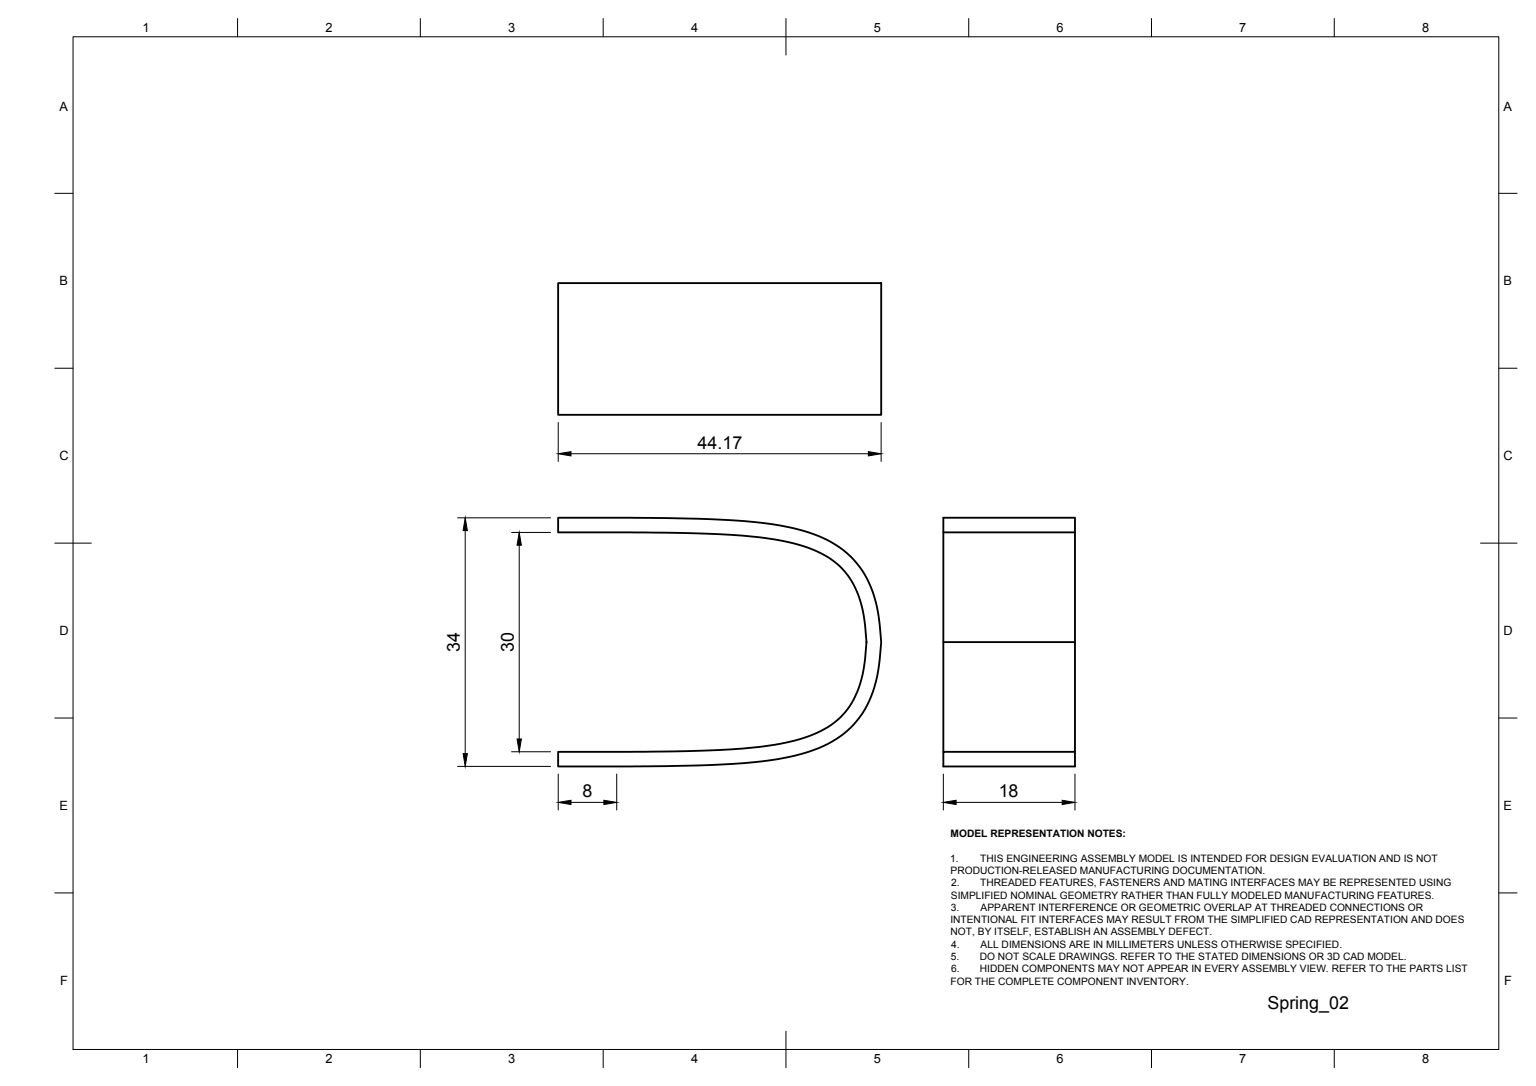
ISO-10303-21;
HEADER;
/* Generated by software containing ST-Developer
 * from STEP Tools, Inc. (www.steptools.com) 
 */

FILE_DESCRIPTION(
/* description */ (''),
/* implementation_level */ '2;1');

FILE_NAME(
/* name */ 'Spring_02.step',
/* time_stamp */ '2026-10-06T13:31:15-07:00',
/* author */ (''),
/* organization */ (''),
/* preprocessor_version */ 'ST-DEVELOPER v20.2',
/* originating_system */ 'Autodesk Translation Framework v15.15.0.0',
/* authorisation */ '');

FILE_SCHEMA (('AUTOMOTIVE_DESIGN { 1 0 10303 214 3 1 1 }'));
ENDSEC;

DATA;
#10=MECHANICAL_DESIGN_GEOMETRIC_PRESENTATION_REPRESENTATION('',(#81),#3154);
#51=B_SPLINE_SURFACE_WITH_KNOTS('',3,1,((#1764,#1765),(#1766,#1767),(#1768,
#1769),(#1770,#1771),(#1772,#1773),(#1774,#1775),(#1776,#1777),(#1778,#1779),
(#1780,#1781),(#1782,#1783),(#1784,#1785),(#1786,#1787),(#1788,#1789),(#1790,
#1791),(#1792,#1793),(#1794,#1795),(#1796,#1797),(#1798,#1799),(#1800,#1801)),
 .UNSPECIFIED.,.F.,.F.,.F.,(4,3,3,3,3,3,4),(2,2),(0.,0.25,0.625,0.869068416619454,
0.996324238316631,1.,1.10633190132162),(0.,2.16230058202055),
 .UNSPECIFIED.);
#52=B_SPLINE_SURFACE_WITH_KNOTS('',5,1,((#1843,#1844),(#1845,#1846),(#1847,
#1848),(#1849,#1850),(#1851,#1852),(#1853,#1854),(#1855,#1856),(#1857,#1858),
(#1859,#1860),(#1861,#1862),(#1863,#1864),(#1865,#1866),(#1867,#1868),(#1869,
#1870),(#1871,#1872),(#1873,#1874),(#1875,#1876),(#1877,#1878),(#1879,#1880),
(#1881,#1882),(#1883,#1884),(#1885,#1886),(#1887,#1888),(#1889,#1890),(#1891,
#1892)),.UNSPECIFIED.,.F.,.F.,.F.,(6,5,1,1,1,1,1,1,1,1,1,1,1,1,1,1,6),(2,
2),(-1.10044937423827,-1.,-0.933333333333333,-0.866666666666667,-0.8,-0.733333333333333,
-0.666666666666667,-0.6,-0.533333333333333,-0.466666666666667,-0.4,-0.333333333333333,
-0.266666666666667,-0.2,-0.133333333333333,-0.0666666666666667,0.),(0.,
2.16),.UNSPECIFIED.);
#53=B_SPLINE_SURFACE_WITH_KNOTS('',5,1,((#2046,#2047),(#2048,#2049),(#2050,
#2051),(#2052,#2053),(#2054,#2055),(#2056,#2057),(#2058,#2059),(#2060,#2061),
(#2062,#2063),(#2064,#2065),(#2066,#2067),(#2068,#2069),(#2070,#2071),(#2072,
#2073),(#2074,#2075),(#2076,#2077),(#2078,#2079),(#2080,#2081),(#2082,#2083),
(#2084,#2085),(#2086,#2087),(#2088,#2089),(#2090,#2091),(#2092,#2093),(#2094,
#2095)),.UNSPECIFIED.,.F.,.F.,.F.,(6,1,1,1,1,1,1,1,1,1,1,1,1,1,1,5,6),(2,
2),(0.,0.0666666666666667,0.133333333333333,0.2,0.266666666666667,0.333333333333333,
0.4,0.466666666666667,0.533333333333333,0.6,0.666666666666667,0.733333333333333,
0.8,0.866666666666667,0.933333333333333,1.,1.10044937423827),(0.,2.16),
 .UNSPECIFIED.);
#54=B_SPLINE_SURFACE_WITH_KNOTS('',3,1,((#2103,#2104),(#2105,#2106),(#2107,
#2108),(#2109,#2110),(#2111,#2112),(#2113,#2114),(#2115,#2116),(#2117,#2118),
(#2119,#2120),(#2121,#2122),(#2123,#2124),(#2125,#2126),(#2127,#2128),(#2129,
#2130),(#2131,#2132),(#2133,#2134),(#2135,#2136),(#2137,#2138),(#2139,#2140)),
 .UNSPECIFIED.,.F.,.F.,.F.,(4,3,3,3,3,3,4),(2,2),(-1.10633190132173,-1.,
-0.996324238316733,-0.869068416619454,-0.625,-0.25,0.),(0.,2.16230058202055),
 .UNSPECIFIED.);
#63=SHAPE_REPRESENTATION_RELATIONSHIP('SRR','None',#3191,#72);
#72=ADVANCED_BREP_SHAPE_REPRESENTATION('',(#90),#3147);
#81=STYLED_ITEM('',(#3243),#90);
#90=MANIFOLD_SOLID_BREP('Body1',#1083);
#102=PLANE('',#1213);
#103=PLANE('',#1214);
#104=PLANE('',#1215);
#105=PLANE('',#1216);
#106=PLANE('',#1217);
#107=PLANE('',#1218);
#108=PLANE('',#1219);
#109=PLANE('',#1220);
#182=FACE_OUTER_BOUND('',#246,.T.);
#183=FACE_OUTER_BOUND('',#247,.T.);
#184=FACE_OUTER_BOUND('',#248,.T.);
#185=FACE_OUTER_BOUND('',#249,.T.);
#186=FACE_OUTER_BOUND('',#250,.T.);
#187=FACE_OUTER_BOUND('',#251,.T.);
#188=FACE_OUTER_BOUND('',#252,.T.);
#189=FACE_OUTER_BOUND('',#253,.T.);
#190=FACE_OUTER_BOUND('',#254,.T.);
#191=FACE_OUTER_BOUND('',#255,.T.);
#192=FACE_OUTER_BOUND('',#256,.T.);
#193=FACE_OUTER_BOUND('',#257,.T.);
#246=EDGE_LOOP('',(#772,#773,#774,#775));
#247=EDGE_LOOP('',(#776,#777,#778,#779));
#248=EDGE_LOOP('',(#780,#781,#782,#783));
#249=EDGE_LOOP('',(#784,#785,#786,#787));
#250=EDGE_LOOP('',(#788,#789,#790,#791));
#251=EDGE_LOOP('',(#792,#793,#794,#795,#796,#797,#798,#799,#800,#801));
#252=EDGE_LOOP('',(#802,#803,#804,#805,#806,#807,#808,#809,#810,#811));
#253=EDGE_LOOP('',(#812,#813,#814,#815));
#254=EDGE_LOOP('',(#816,#817,#818,#819));
#255=EDGE_LOOP('',(#820,#821,#822,#823));
#256=EDGE_LOOP('',(#824,#825,#826,#827));
#257=EDGE_LOOP('',(#828,#829,#830,#831));
#308=LINE('',#1746,#374);
#309=LINE('',#1748,#375);
#310=LINE('',#1750,#376);
#311=LINE('',#1751,#377);
#312=LINE('',#1755,#378);
#313=LINE('',#1756,#379);
#314=LINE('',#1757,#380);
#315=LINE('',#1761,#381);
#316=LINE('',#1762,#382);
#317=LINE('',#1763,#383);
#318=LINE('',#1804,#384);
#319=LINE('',#1919,#385);
#320=LINE('',#1966,#386);
#321=LINE('',#1968,#387);
#322=LINE('',#1970,#388);
#323=LINE('',#2022,#389);
#324=LINE('',#2024,#390);
#325=LINE('',#2026,#391);
#326=LINE('',#2096,#392);
#327=LINE('',#2098,#393);
#328=LINE('',#2100,#394);
#329=LINE('',#2102,#395);
#374=VECTOR('',#1342,10.);
#375=VECTOR('',#1343,10.);
#376=VECTOR('',#1344,10.);
#377=VECTOR('',#1345,10.);
#378=VECTOR('',#1348,10.);
#379=VECTOR('',#1349,10.);
#380=VECTOR('',#1350,10.);
#381=VECTOR('',#1353,10.);
#382=VECTOR('',#1354,10.);
#383=VECTOR('',#1355,10.);
#384=VECTOR('',#1356,10.);
#385=VECTOR('',#1357,10.);
#386=VECTOR('',#1360,10.);
#387=VECTOR('',#1361,10.);
#388=VECTOR('',#1362,10.);
#389=VECTOR('',#1365,10.);
#390=VECTOR('',#1366,10.);
#391=VECTOR('',#1367,10.);
#392=VECTOR('',#1368,10.);
#393=VECTOR('',#1371,10.);
#394=VECTOR('',#1374,10.);
#395=VECTOR('',#1377,10.);
#442=B_SPLINE_CURVE_WITH_KNOTS('',3,(#1805,#1806,#1807,#1808,#1809,#1810,
#1811,#1812,#1813,#1814,#1815,#1816,#1817,#1818,#1819,#1820,#1821,#1822,
#1823),.UNSPECIFIED.,.F.,.F.,(4,3,3,3,3,3,4),(0.,0.25,0.625,0.869068416619454,
0.996324238316631,1.,1.03680973061555),.UNSPECIFIED.);
#443=B_SPLINE_CURVE_WITH_KNOTS('',3,(#1824,#1825,#1826,#1827,#1828,#1829,
#1830,#1831,#1832,#1833,#1834,#1835,#1836,#1837,#1838,#1839,#1840,#1841,
#1842),.UNSPECIFIED.,.F.,.F.,(4,3,3,3,3,3,4),(-1.03680973061555,-1.,-0.996324238316631,
-0.869068416619454,-0.625,-0.25,0.),.UNSPECIFIED.);
#444=B_SPLINE_CURVE_WITH_KNOTS('',5,(#1894,#1895,#1896,#1897,#1898,#1899,
#1900,#1901,#1902,#1903,#1904,#1905,#1906,#1907,#1908,#1909,#1910,#1911,
#1912,#1913,#1914,#1915,#1916,#1917),.UNSPECIFIED.,.F.,.F.,(6,1,1,1,1,1,
1,1,1,1,1,1,1,1,1,4,6),(0.,0.0666666666666667,0.133333333333333,0.2,0.266666666666667,
0.333333333333333,0.4,0.466666666666667,0.533333333333333,0.6,0.666666666666667,
0.733333333333333,0.8,0.866666666666667,0.933333333333333,1.,1.04017974969531),
 .UNSPECIFIED.);
#445=B_SPLINE_CURVE_WITH_KNOTS('',5,(#1920,#1921,#1922,#1923,#1924,#1925,
#1926,#1927,#1928,#1929,#1930,#1931,#1932,#1933,#1934,#1935,#1936,#1937,
#1938,#1939,#1940,#1941,#1942,#1943),.UNSPECIFIED.,.F.,.F.,(6,1,1,1,1,1,
1,1,1,1,1,1,1,1,1,4,6),(0.,0.0666666666666667,0.133333333333333,0.2,0.266666666666667,
0.333333333333333,0.4,0.466666666666667,0.533333333333333,0.6,0.666666666666667,
0.733333333333333,0.8,0.866666666666667,0.933333333333333,1.,1.04017974969531),
 .UNSPECIFIED.);
#446=B_SPLINE_CURVE_WITH_KNOTS('',3,(#1946,#1947,#1948,#1949,#1950,#1951,
#1952,#1953,#1954,#1955,#1956,#1957,#1958,#1959,#1960,#1961,#1962,#1963,
#1964),.UNSPECIFIED.,.F.,.F.,(4,3,3,3,3,3,4),(-1.03680973061555,-1.,-0.996324238316733,
-0.869068416619454,-0.625,-0.25,0.),.UNSPECIFIED.);
#447=B_SPLINE_CURVE_WITH_KNOTS('',5,(#1971,#1972,#1973,#1974,#1975,#1976,
#1977,#1978,#1979,#1980,#1981,#1982,#1983,#1984,#1985,#1986,#1987,#1988,
#1989,#1990,#1991,#1992,#1993,#1994),.UNSPECIFIED.,.F.,.F.,(6,4,1,1,1,1,
1,1,1,1,1,1,1,1,1,1,6),(-1.04017974969531,-1.,-0.933333333333333,-0.866666666666667,
-0.8,-0.733333333333333,-0.666666666666667,-0.6,-0.533333333333333,-0.466666666666667,
-0.4,-0.333333333333333,-0.266666666666667,-0.2,-0.133333333333333,-0.0666666666666667,
0.),.UNSPECIFIED.);
#448=B_SPLINE_CURVE_WITH_KNOTS('',5,(#1997,#1998,#1999,#2000,#2001,#2002,
#2003,#2004,#2005,#2006,#2007,#2008,#2009,#2010,#2011,#2012,#2013,#2014,
#2015,#2016,#2017,#2018,#2019,#2020),.UNSPECIFIED.,.F.,.F.,(6,4,1,1,1,1,
1,1,1,1,1,1,1,1,1,1,6),(-1.04017974969531,-1.,-0.933333333333333,-0.866666666666667,
-0.8,-0.733333333333333,-0.666666666666667,-0.6,-0.533333333333333,-0.466666666666667,
-0.4,-0.333333333333333,-0.266666666666667,-0.2,-0.133333333333333,-0.0666666666666667,
0.),.UNSPECIFIED.);
#449=B_SPLINE_CURVE_WITH_KNOTS('',3,(#2027,#2028,#2029,#2030,#2031,#2032,
#2033,#2034,#2035,#2036,#2037,#2038,#2039,#2040,#2041,#2042,#2043,#2044,
#2045),.UNSPECIFIED.,.F.,.F.,(4,3,3,3,3,3,4),(0.,0.25,0.625,0.869068416619454,
0.996324238316733,1.,1.03680973061555),.UNSPECIFIED.);
#496=VERTEX_POINT('',#1744);
#497=VERTEX_POINT('',#1745);
#498=VERTEX_POINT('',#1747);
#499=VERTEX_POINT('',#1749);
#500=VERTEX_POINT('',#1753);
#501=VERTEX_POINT('',#1754);
#502=VERTEX_POINT('',#1759);
#503=VERTEX_POINT('',#1760);
#504=VERTEX_POINT('',#1802);
#505=VERTEX_POINT('',#1803);
#506=VERTEX_POINT('',#1893);
#507=VERTEX_POINT('',#1918);
#508=VERTEX_POINT('',#1945);
#509=VERTEX_POINT('',#1965);
#510=VERTEX_POINT('',#1967);
#511=VERTEX_POINT('',#1969);
#512=VERTEX_POINT('',#1996);
#513=VERTEX_POINT('',#2021);
#514=VERTEX_POINT('',#2023);
#515=VERTEX_POINT('',#2025);
#602=EDGE_CURVE('',#496,#497,#308,.T.);
#603=EDGE_CURVE('',#498,#497,#309,.T.);
#604=EDGE_CURVE('',#498,#499,#310,.T.);
#605=EDGE_CURVE('',#496,#499,#311,.T.);
#606=EDGE_CURVE('',#500,#501,#312,.T.);
#607=EDGE_CURVE('',#497,#501,#313,.T.);
#608=EDGE_CURVE('',#500,#496,#314,.T.);
#609=EDGE_CURVE('',#502,#503,#315,.T.);
#610=EDGE_CURVE('',#501,#503,#316,.T.);
#611=EDGE_CURVE('',#502,#500,#317,.T.);
#612=EDGE_CURVE('',#504,#505,#318,.F.);
#613=EDGE_CURVE('',#503,#505,#442,.T.);
#614=EDGE_CURVE('',#504,#502,#443,.T.);
#615=EDGE_CURVE('',#506,#498,#444,.F.);
#616=EDGE_CURVE('',#507,#506,#319,.F.);
#617=EDGE_CURVE('',#499,#507,#445,.T.);
#618=EDGE_CURVE('',#505,#508,#446,.T.);
#619=EDGE_CURVE('',#508,#509,#320,.T.);
#620=EDGE_CURVE('',#509,#510,#321,.T.);
#621=EDGE_CURVE('',#510,#511,#322,.T.);
#622=EDGE_CURVE('',#511,#506,#447,.F.);
#623=EDGE_CURVE('',#507,#512,#448,.T.);
#624=EDGE_CURVE('',#512,#513,#323,.T.);
#625=EDGE_CURVE('',#513,#514,#324,.T.);
#626=EDGE_CURVE('',#514,#515,#325,.T.);
#627=EDGE_CURVE('',#515,#504,#449,.T.);
#628=EDGE_CURVE('',#512,#511,#326,.T.);
#629=EDGE_CURVE('',#513,#510,#327,.T.);
#630=EDGE_CURVE('',#514,#509,#328,.T.);
#631=EDGE_CURVE('',#515,#508,#329,.T.);
#772=ORIENTED_EDGE('',*,*,#602,.T.);
#773=ORIENTED_EDGE('',*,*,#603,.F.);
#774=ORIENTED_EDGE('',*,*,#604,.T.);
#775=ORIENTED_EDGE('',*,*,#605,.F.);
#776=ORIENTED_EDGE('',*,*,#606,.T.);
#777=ORIENTED_EDGE('',*,*,#607,.F.);
#778=ORIENTED_EDGE('',*,*,#602,.F.);
#779=ORIENTED_EDGE('',*,*,#608,.F.);
#780=ORIENTED_EDGE('',*,*,#609,.T.);
#781=ORIENTED_EDGE('',*,*,#610,.F.);
#782=ORIENTED_EDGE('',*,*,#606,.F.);
#783=ORIENTED_EDGE('',*,*,#611,.F.);
#784=ORIENTED_EDGE('',*,*,#612,.T.);
#785=ORIENTED_EDGE('',*,*,#613,.F.);
#786=ORIENTED_EDGE('',*,*,#609,.F.);
#787=ORIENTED_EDGE('',*,*,#614,.F.);
#788=ORIENTED_EDGE('',*,*,#604,.F.);
#789=ORIENTED_EDGE('',*,*,#615,.F.);
#790=ORIENTED_EDGE('',*,*,#616,.F.);
#791=ORIENTED_EDGE('',*,*,#617,.F.);
#792=ORIENTED_EDGE('',*,*,#618,.T.);
#793=ORIENTED_EDGE('',*,*,#619,.T.);
#794=ORIENTED_EDGE('',*,*,#620,.T.);
#795=ORIENTED_EDGE('',*,*,#621,.T.);
#796=ORIENTED_EDGE('',*,*,#622,.T.);
#797=ORIENTED_EDGE('',*,*,#615,.T.);
#798=ORIENTED_EDGE('',*,*,#603,.T.);
#799=ORIENTED_EDGE('',*,*,#607,.T.);
#800=ORIENTED_EDGE('',*,*,#610,.T.);
#801=ORIENTED_EDGE('',*,*,#613,.T.);
#802=ORIENTED_EDGE('',*,*,#623,.T.);
#803=ORIENTED_EDGE('',*,*,#624,.T.);
#804=ORIENTED_EDGE('',*,*,#625,.T.);
#805=ORIENTED_EDGE('',*,*,#626,.T.);
#806=ORIENTED_EDGE('',*,*,#627,.T.);
#807=ORIENTED_EDGE('',*,*,#614,.T.);
#808=ORIENTED_EDGE('',*,*,#611,.T.);
#809=ORIENTED_EDGE('',*,*,#608,.T.);
#810=ORIENTED_EDGE('',*,*,#605,.T.);
#811=ORIENTED_EDGE('',*,*,#617,.T.);
#812=ORIENTED_EDGE('',*,*,#616,.T.);
#813=ORIENTED_EDGE('',*,*,#622,.F.);
#814=ORIENTED_EDGE('',*,*,#628,.F.);
#815=ORIENTED_EDGE('',*,*,#623,.F.);
#816=ORIENTED_EDGE('',*,*,#628,.T.);
#817=ORIENTED_EDGE('',*,*,#621,.F.);
#818=ORIENTED_EDGE('',*,*,#629,.F.);
#819=ORIENTED_EDGE('',*,*,#624,.F.);
#820=ORIENTED_EDGE('',*,*,#629,.T.);
#821=ORIENTED_EDGE('',*,*,#620,.F.);
#822=ORIENTED_EDGE('',*,*,#630,.F.);
#823=ORIENTED_EDGE('',*,*,#625,.F.);
#824=ORIENTED_EDGE('',*,*,#630,.T.);
#825=ORIENTED_EDGE('',*,*,#619,.F.);
#826=ORIENTED_EDGE('',*,*,#631,.F.);
#827=ORIENTED_EDGE('',*,*,#626,.F.);
#828=ORIENTED_EDGE('',*,*,#631,.T.);
#829=ORIENTED_EDGE('',*,*,#618,.F.);
#830=ORIENTED_EDGE('',*,*,#612,.F.);
#831=ORIENTED_EDGE('',*,*,#627,.F.);
#1033=ADVANCED_FACE('',(#182),#102,.T.);
#1034=ADVANCED_FACE('',(#183),#103,.T.);
#1035=ADVANCED_FACE('',(#184),#104,.T.);
#1036=ADVANCED_FACE('',(#185),#51,.T.);
#1037=ADVANCED_FACE('',(#186),#52,.T.);
#1038=ADVANCED_FACE('',(#187),#105,.T.);
#1039=ADVANCED_FACE('',(#188),#106,.F.);
#1040=ADVANCED_FACE('',(#189),#53,.T.);
#1041=ADVANCED_FACE('',(#190),#107,.T.);
#1042=ADVANCED_FACE('',(#191),#108,.T.);
#1043=ADVANCED_FACE('',(#192),#109,.T.);
#1044=ADVANCED_FACE('',(#193),#54,.T.);
#1083=CLOSED_SHELL('',(#1033,#1034,#1035,#1036,#1037,#1038,#1039,#1040,
#1041,#1042,#1043,#1044));
#1212=AXIS2_PLACEMENT_3D('',#1742,#1338,#1339);
#1213=AXIS2_PLACEMENT_3D('',#1743,#1340,#1341);
#1214=AXIS2_PLACEMENT_3D('',#1752,#1346,#1347);
#1215=AXIS2_PLACEMENT_3D('',#1758,#1351,#1352);
#1216=AXIS2_PLACEMENT_3D('',#1944,#1358,#1359);
#1217=AXIS2_PLACEMENT_3D('',#1995,#1363,#1364);
#1218=AXIS2_PLACEMENT_3D('',#2097,#1369,#1370);
#1219=AXIS2_PLACEMENT_3D('',#2099,#1372,#1373);
#1220=AXIS2_PLACEMENT_3D('',#2101,#1375,#1376);
#1338=DIRECTION('axis',(0.,0.,1.));
#1339=DIRECTION('refdir',(1.,0.,0.));
#1340=DIRECTION('center_axis',(-1.,0.,0.));
#1341=DIRECTION('ref_axis',(0.,0.,1.));
#1342=DIRECTION('',(0.,1.,0.));
#1343=DIRECTION('',(0.,0.,1.));
#1344=DIRECTION('',(0.,-1.,0.));
#1345=DIRECTION('',(0.,0.,-1.));
#1346=DIRECTION('center_axis',(0.,0.,1.));
#1347=DIRECTION('ref_axis',(1.,0.,0.));
#1348=DIRECTION('',(0.,1.,0.));
#1349=DIRECTION('',(1.,0.,0.));
#1350=DIRECTION('',(-1.,0.,0.));
#1351=DIRECTION('center_axis',(1.,0.,0.));
#1352=DIRECTION('ref_axis',(0.,0.,-1.));
#1353=DIRECTION('',(0.,1.,0.));
#1354=DIRECTION('',(0.,0.,-1.));
#1355=DIRECTION('',(0.,0.,1.));
#1356=DIRECTION('',(0.,-1.,0.));
#1357=DIRECTION('',(0.,-1.,0.));
#1358=DIRECTION('center_axis',(0.,1.,0.));
#1359=DIRECTION('ref_axis',(1.,0.,0.));
#1360=DIRECTION('',(0.,0.,1.));
#1361=DIRECTION('',(1.,0.,0.));
#1362=DIRECTION('',(0.,0.,-1.));
#1363=DIRECTION('center_axis',(0.,1.,0.));
#1364=DIRECTION('ref_axis',(1.,0.,0.));
#1365=DIRECTION('',(0.,0.,1.));
#1366=DIRECTION('',(-1.,0.,0.));
#1367=DIRECTION('',(0.,0.,-1.));
#1368=DIRECTION('',(0.,1.,0.));
#1369=DIRECTION('center_axis',(1.,0.,0.));
#1370=DIRECTION('ref_axis',(0.,0.,-1.));
#1371=DIRECTION('',(0.,1.,0.));
#1372=DIRECTION('center_axis',(0.,0.,1.));
#1373=DIRECTION('ref_axis',(1.,0.,0.));
#1374=DIRECTION('',(0.,1.,0.));
#1375=DIRECTION('center_axis',(-1.,0.,0.));
#1376=DIRECTION('ref_axis',(0.,0.,1.));
#1377=DIRECTION('',(0.,1.,0.));
#1742=CARTESIAN_POINT('',(0.,0.,0.));
#1743=CARTESIAN_POINT('Origin',(-17.,0.,316.));
#1744=CARTESIAN_POINT('',(-17.,-9.,324.));
#1745=CARTESIAN_POINT('',(-17.,9.,324.));
#1746=CARTESIAN_POINT('',(-17.,0.,324.));
#1747=CARTESIAN_POINT('',(-17.,9.,316.));
#1748=CARTESIAN_POINT('',(-17.,9.,324.));
#1749=CARTESIAN_POINT('',(-17.,-9.,316.));
#1750=CARTESIAN_POINT('',(-17.,0.,316.));
#1751=CARTESIAN_POINT('',(-17.,-9.,324.));
#1752=CARTESIAN_POINT('Origin',(-17.,0.,324.));
#1753=CARTESIAN_POINT('',(-15.,-9.,324.));
#1754=CARTESIAN_POINT('',(-15.,9.,324.));
#1755=CARTESIAN_POINT('',(-15.,0.,324.));
#1756=CARTESIAN_POINT('',(-17.,9.,324.));
#1757=CARTESIAN_POINT('',(-17.,-9.,324.));
#1758=CARTESIAN_POINT('Origin',(-15.,0.,324.));
#1759=CARTESIAN_POINT('',(-15.,-9.,316.));
#1760=CARTESIAN_POINT('',(-15.,9.,316.));
#1761=CARTESIAN_POINT('',(-15.,0.,316.));
#1762=CARTESIAN_POINT('',(-15.,9.,324.));
#1763=CARTESIAN_POINT('',(-15.,-9.,324.));
#1764=CARTESIAN_POINT('Ctrl Pts',(-15.,-9.01917151683795,316.));
#1765=CARTESIAN_POINT('Ctrl Pts',(-15.,12.6038343033676,316.));
#1766=CARTESIAN_POINT('Ctrl Pts',(-15.,-9.01917151683795,312.917218954967));
#1767=CARTESIAN_POINT('Ctrl Pts',(-15.,12.6038343033676,312.917218954967));
#1768=CARTESIAN_POINT('Ctrl Pts',(-14.9804665025967,-9.01917151683795,309.284971969759));
#1769=CARTESIAN_POINT('Ctrl Pts',(-14.9804665025967,12.6038343033676,309.284971969759));
#1770=CARTESIAN_POINT('Ctrl Pts',(-14.8743203079702,-9.01917151683795,305.389849883143));
#1771=CARTESIAN_POINT('Ctrl Pts',(-14.8743203079702,12.6038343033676,305.389849883143));
#1772=CARTESIAN_POINT('Ctrl Pts',(-14.7151010160305,-9.01917151683795,299.547166753218));
#1773=CARTESIAN_POINT('Ctrl Pts',(-14.7151010160305,12.6038343033676,299.547166753218));
#1774=CARTESIAN_POINT('Ctrl Pts',(-14.3613339472215,-9.01917151683795,293.114195242939));
#1775=CARTESIAN_POINT('Ctrl Pts',(-14.3613339472215,12.6038343033676,293.114195242939));
#1776=CARTESIAN_POINT('Ctrl Pts',(-12.5329121501934,-9.01917151683795,288.887907445925));
#1777=CARTESIAN_POINT('Ctrl Pts',(-12.5329121501934,12.6038343033676,288.887907445925));
#1778=CARTESIAN_POINT('Ctrl Pts',(-11.3428854490917,-9.01917151683795,286.13723179047));
#1779=CARTESIAN_POINT('Ctrl Pts',(-11.3428854490917,12.6038343033676,286.13723179047));
#1780=CARTESIAN_POINT('Ctrl Pts',(-9.6259837213127,-9.01917151683795,284.320800585332));
#1781=CARTESIAN_POINT('Ctrl Pts',(-9.6259837213127,12.6038343033676,284.320800585332));
#1782=CARTESIAN_POINT('Ctrl Pts',(-6.96718239188881,-9.01917151683795,283.179505866003));
#1783=CARTESIAN_POINT('Ctrl Pts',(-6.96718239188881,12.6038343033676,283.179505866003));
#1784=CARTESIAN_POINT('Ctrl Pts',(-5.58089918248474,-9.01917151683795,282.584441583133));
#1785=CARTESIAN_POINT('Ctrl Pts',(-5.58089918248474,12.6038343033676,282.584441583133));
#1786=CARTESIAN_POINT('Ctrl Pts',(-3.9277760249776,-9.01917151683795,282.184209001161));
#1787=CARTESIAN_POINT('Ctrl Pts',(-3.9277760249776,12.6038343033676,282.184209001161));
#1788=CARTESIAN_POINT('Ctrl Pts',(-2.00000000000228,-9.01917151683795,282.007690234858));
#1789=CARTESIAN_POINT('Ctrl Pts',(-2.00000000000228,12.6038343033676,282.007690234858));
#1790=CARTESIAN_POINT('Ctrl Pts',(-1.94431052069769,-9.01917151683795,282.002590971222));
#1791=CARTESIAN_POINT('Ctrl Pts',(-1.94431052069769,12.6038343033676,282.002590971222));
#1792=CARTESIAN_POINT('Ctrl Pts',(-1.88839473154277,-9.01917151683795,281.997678278411));
#1793=CARTESIAN_POINT('Ctrl Pts',(-1.88839473154277,12.6038343033676,281.997678278411));
#1794=CARTESIAN_POINT('Ctrl Pts',(-1.8322528584517,-9.01917151683795,281.992952808398));
#1795=CARTESIAN_POINT('Ctrl Pts',(-1.8322528584517,12.6038343033676,281.992952808398));
#1796=CARTESIAN_POINT('Ctrl Pts',(-0.067982678772372,-9.01917151683795,
281.844453918553));
#1797=CARTESIAN_POINT('Ctrl Pts',(-0.067982678772372,12.6038343033676,281.844453918553));
#1798=CARTESIAN_POINT('Ctrl Pts',(1.69628750090713,-9.01917151683795,281.695955028709));
#1799=CARTESIAN_POINT('Ctrl Pts',(1.69628750090713,12.6038343033676,281.695955028709));
#1800=CARTESIAN_POINT('Ctrl Pts',(3.46055768058644,-9.01917151683795,281.547456138864));
#1801=CARTESIAN_POINT('Ctrl Pts',(3.46055768058644,12.6038343033676,281.547456138864));
#1802=CARTESIAN_POINT('',(-2.61075883134509E-14,-9.,281.838731806123));
#1803=CARTESIAN_POINT('',(-2.61075883134509E-14,9.,281.838731806123));
#1804=CARTESIAN_POINT('',(-5.91540705308091E-14,9.,281.838731806123));
#1805=CARTESIAN_POINT('Ctrl Pts',(-15.,9.,316.));
#1806=CARTESIAN_POINT('Ctrl Pts',(-15.,9.,312.917218954967));
#1807=CARTESIAN_POINT('Ctrl Pts',(-14.9804665025967,9.,309.284971969759));
#1808=CARTESIAN_POINT('Ctrl Pts',(-14.8743203079702,9.,305.389849883143));
#1809=CARTESIAN_POINT('Ctrl Pts',(-14.7151010160305,9.,299.547166753218));
#1810=CARTESIAN_POINT('Ctrl Pts',(-14.3613339472215,9.,293.114195242939));
#1811=CARTESIAN_POINT('Ctrl Pts',(-12.5329121501934,9.,288.887907445925));
#1812=CARTESIAN_POINT('Ctrl Pts',(-11.3428854490917,9.,286.13723179047));
#1813=CARTESIAN_POINT('Ctrl Pts',(-9.6259837213127,9.,284.320800585332));
#1814=CARTESIAN_POINT('Ctrl Pts',(-6.96718239188881,9.,283.179505866003));
#1815=CARTESIAN_POINT('Ctrl Pts',(-5.58089918248474,9.,282.584441583133));
#1816=CARTESIAN_POINT('Ctrl Pts',(-3.9277760249776,9.,282.184209001161));
#1817=CARTESIAN_POINT('Ctrl Pts',(-2.00000000000228,9.,282.007690234858));
#1818=CARTESIAN_POINT('Ctrl Pts',(-1.94431052069769,9.,282.002590971222));
#1819=CARTESIAN_POINT('Ctrl Pts',(-1.88839473154277,9.,281.997678278411));
#1820=CARTESIAN_POINT('Ctrl Pts',(-1.8322528584517,9.,281.992952808398));
#1821=CARTESIAN_POINT('Ctrl Pts',(-1.22150190563454,9.,281.941545807639));
#1822=CARTESIAN_POINT('Ctrl Pts',(-0.610750952817352,9.,281.890138806881));
#1823=CARTESIAN_POINT('Ctrl Pts',(-1.61426427780498E-13,9.,281.838731806122));
#1824=CARTESIAN_POINT('Ctrl Pts',(-1.39499523044151E-13,-9.,281.838731806122));
#1825=CARTESIAN_POINT('Ctrl Pts',(-0.610750952817337,-9.,281.890138806881));
#1826=CARTESIAN_POINT('Ctrl Pts',(-1.22150190563453,-9.,281.941545807639));
#1827=CARTESIAN_POINT('Ctrl Pts',(-1.8322528584517,-9.,281.992952808398));
#1828=CARTESIAN_POINT('Ctrl Pts',(-1.88839473154277,-9.,281.997678278411));
#1829=CARTESIAN_POINT('Ctrl Pts',(-1.94431052069769,-9.,282.002590971222));
#1830=CARTESIAN_POINT('Ctrl Pts',(-2.00000000000228,-9.,282.007690234858));
#1831=CARTESIAN_POINT('Ctrl Pts',(-3.9277760249776,-9.,282.184209001161));
#1832=CARTESIAN_POINT('Ctrl Pts',(-5.58089918248474,-9.,282.584441583133));
#1833=CARTESIAN_POINT('Ctrl Pts',(-6.96718239188881,-9.,283.179505866003));
#1834=CARTESIAN_POINT('Ctrl Pts',(-9.6259837213127,-9.,284.320800585332));
#1835=CARTESIAN_POINT('Ctrl Pts',(-11.3428854490917,-9.,286.13723179047));
#1836=CARTESIAN_POINT('Ctrl Pts',(-12.5329121501934,-9.,288.887907445925));
#1837=CARTESIAN_POINT('Ctrl Pts',(-14.3613339472215,-9.,293.114195242939));
#1838=CARTESIAN_POINT('Ctrl Pts',(-14.7151010160305,-9.,299.547166753218));
#1839=CARTESIAN_POINT('Ctrl Pts',(-14.8743203079702,-9.,305.389849883143));
#1840=CARTESIAN_POINT('Ctrl Pts',(-14.9804665025967,-9.,309.284971969759));
#1841=CARTESIAN_POINT('Ctrl Pts',(-15.,-9.,312.917218954967));
#1842=CARTESIAN_POINT('Ctrl Pts',(-15.,-9.,316.));
#1843=CARTESIAN_POINT('Ctrl Pts',(3.,-9.,279.579149238152));
#1844=CARTESIAN_POINT('Ctrl Pts',(3.,12.6,279.579149238152));
#1845=CARTESIAN_POINT('Ctrl Pts',(2.,-9.,279.663319390522));
#1846=CARTESIAN_POINT('Ctrl Pts',(2.,12.6,279.663319390522));
#1847=CARTESIAN_POINT('Ctrl Pts',(1.,-9.,279.747489542891));
#1848=CARTESIAN_POINT('Ctrl Pts',(1.,12.6,279.747489542891));
#1849=CARTESIAN_POINT('Ctrl Pts',(-5.55111512312578E-16,-9.,279.831659695261));
#1850=CARTESIAN_POINT('Ctrl Pts',(-5.55111512312578E-16,12.6,279.831659695261));
#1851=CARTESIAN_POINT('Ctrl Pts',(-1.,-9.,279.91582984763));
#1852=CARTESIAN_POINT('Ctrl Pts',(-1.,12.6,279.91582984763));
#1853=CARTESIAN_POINT('Ctrl Pts',(-2.,-9.,280.));
#1854=CARTESIAN_POINT('Ctrl Pts',(-2.,12.6,280.));
#1855=CARTESIAN_POINT('Ctrl Pts',(-2.66368424066569,-9.,280.055862403662));
#1856=CARTESIAN_POINT('Ctrl Pts',(-2.66368424066569,12.6,280.055862403662));
#1857=CARTESIAN_POINT('Ctrl Pts',(-3.9517913938126,-9.,280.208504145521));
#1858=CARTESIAN_POINT('Ctrl Pts',(-3.9517913938126,12.6,280.208504145521));
#1859=CARTESIAN_POINT('Ctrl Pts',(-5.76616670029465,-9.,280.560219196132));
#1860=CARTESIAN_POINT('Ctrl Pts',(-5.76616670029465,12.6,280.560219196132));
#1861=CARTESIAN_POINT('Ctrl Pts',(-7.94806288019228,-9.,281.276448102944));
#1862=CARTESIAN_POINT('Ctrl Pts',(-7.94806288019228,12.6,281.276448102944));
#1863=CARTESIAN_POINT('Ctrl Pts',(-10.2723403348262,-9.,282.590975648728));
#1864=CARTESIAN_POINT('Ctrl Pts',(-10.2723403348262,12.6,282.590975648728));
#1865=CARTESIAN_POINT('Ctrl Pts',(-12.1890242800701,-9.,284.326851421562));
#1866=CARTESIAN_POINT('Ctrl Pts',(-12.1890242800701,12.6,284.326851421562));
#1867=CARTESIAN_POINT('Ctrl Pts',(-13.7033484644208,-9.,286.473438815185));
#1868=CARTESIAN_POINT('Ctrl Pts',(-13.7033484644208,12.6,286.473438815185));
#1869=CARTESIAN_POINT('Ctrl Pts',(-14.8403951587419,-9.,288.995763819941));
#1870=CARTESIAN_POINT('Ctrl Pts',(-14.8403951587419,12.6,288.995763819941));
#1871=CARTESIAN_POINT('Ctrl Pts',(-15.6496061172615,-9.,291.82914277586));
#1872=CARTESIAN_POINT('Ctrl Pts',(-15.6496061172615,12.6,291.82914277586));
#1873=CARTESIAN_POINT('Ctrl Pts',(-16.1926929497518,-9.,294.892205598351));
#1874=CARTESIAN_POINT('Ctrl Pts',(-16.1926929497518,12.6,294.892205598351));
#1875=CARTESIAN_POINT('Ctrl Pts',(-16.5359735439045,-9.,298.095070696299));
#1876=CARTESIAN_POINT('Ctrl Pts',(-16.5359735439045,12.6,298.095070696299));
#1877=CARTESIAN_POINT('Ctrl Pts',(-16.7422790149997,-9.,301.348120547886));
#1878=CARTESIAN_POINT('Ctrl Pts',(-16.7422790149997,12.6,301.348120547886));
#1879=CARTESIAN_POINT('Ctrl Pts',(-16.8634487703245,-9.,304.57015716772));
#1880=CARTESIAN_POINT('Ctrl Pts',(-16.8634487703245,12.6,304.57015716772));
#1881=CARTESIAN_POINT('Ctrl Pts',(-16.9338349467122,-9.,307.69587590639));
#1882=CARTESIAN_POINT('Ctrl Pts',(-16.9338349467122,12.6,307.69587590639));
#1883=CARTESIAN_POINT('Ctrl Pts',(-16.9745170477256,-9.,310.674187150777));
#1884=CARTESIAN_POINT('Ctrl Pts',(-16.9745170477256,12.6,310.674187150777));
#1885=CARTESIAN_POINT('Ctrl Pts',(-16.9920318646118,-9.,312.909176752281));
#1886=CARTESIAN_POINT('Ctrl Pts',(-16.9920318646118,12.6,312.909176752281));
#1887=CARTESIAN_POINT('Ctrl Pts',(-16.9985513080952,-9.,314.491917916066));
#1888=CARTESIAN_POINT('Ctrl Pts',(-16.9985513080952,12.6,314.491917916066));
#1889=CARTESIAN_POINT('Ctrl Pts',(-17.,-9.,315.50441646936));
#1890=CARTESIAN_POINT('Ctrl Pts',(-17.,12.6,315.50441646936));
#1891=CARTESIAN_POINT('Ctrl Pts',(-17.,-9.,316.));
#1892=CARTESIAN_POINT('Ctrl Pts',(-17.,12.6,316.));
#1893=CARTESIAN_POINT('',(-1.13335267097151E-15,9.,279.831659695261));
#1894=CARTESIAN_POINT('Ctrl Pts',(-17.,9.,316.));
#1895=CARTESIAN_POINT('Ctrl Pts',(-17.,9.,315.50441646936));
#1896=CARTESIAN_POINT('Ctrl Pts',(-16.9985513080952,9.,314.491917916066));
#1897=CARTESIAN_POINT('Ctrl Pts',(-16.9920318646118,9.,312.909176752281));
#1898=CARTESIAN_POINT('Ctrl Pts',(-16.9745170477256,9.,310.674187150777));
#1899=CARTESIAN_POINT('Ctrl Pts',(-16.9338349467122,9.,307.69587590639));
#1900=CARTESIAN_POINT('Ctrl Pts',(-16.8634487703245,9.,304.57015716772));
#1901=CARTESIAN_POINT('Ctrl Pts',(-16.7422790149997,9.,301.348120547886));
#1902=CARTESIAN_POINT('Ctrl Pts',(-16.5359735439045,9.,298.095070696299));
#1903=CARTESIAN_POINT('Ctrl Pts',(-16.1926929497518,9.,294.892205598351));
#1904=CARTESIAN_POINT('Ctrl Pts',(-15.6496061172615,9.,291.82914277586));
#1905=CARTESIAN_POINT('Ctrl Pts',(-14.8403951587419,9.,288.995763819941));
#1906=CARTESIAN_POINT('Ctrl Pts',(-13.7033484644208,9.,286.473438815185));
#1907=CARTESIAN_POINT('Ctrl Pts',(-12.1890242800701,9.,284.326851421562));
#1908=CARTESIAN_POINT('Ctrl Pts',(-10.2723403348262,9.,282.590975648728));
#1909=CARTESIAN_POINT('Ctrl Pts',(-7.94806288019228,9.,281.276448102944));
#1910=CARTESIAN_POINT('Ctrl Pts',(-5.76616670029465,9.,280.560219196132));
#1911=CARTESIAN_POINT('Ctrl Pts',(-3.9517913938126,9.,280.208504145521));
#1912=CARTESIAN_POINT('Ctrl Pts',(-2.66368424066569,9.,280.055862403662));
#1913=CARTESIAN_POINT('Ctrl Pts',(-1.60000000000001,9.,279.966331939052));
#1914=CARTESIAN_POINT('Ctrl Pts',(-1.20000000000001,9.,279.932663878104));
#1915=CARTESIAN_POINT('Ctrl Pts',(-0.800000000000013,9.,279.898995817156));
#1916=CARTESIAN_POINT('Ctrl Pts',(-0.400000000000013,9.,279.865327756209));
#1917=CARTESIAN_POINT('Ctrl Pts',(-2.04350425470068E-14,9.,279.831659695261));
#1918=CARTESIAN_POINT('',(-1.04083408558608E-15,-9.,279.831659695261));
#1919=CARTESIAN_POINT('',(-3.40005801291454E-15,9.,279.831659695261));
#1920=CARTESIAN_POINT('Ctrl Pts',(-17.,-9.,316.));
#1921=CARTESIAN_POINT('Ctrl Pts',(-17.,-9.,315.50441646936));
#1922=CARTESIAN_POINT('Ctrl Pts',(-16.9985513080952,-9.,314.491917916066));
#1923=CARTESIAN_POINT('Ctrl Pts',(-16.9920318646118,-9.,312.909176752281));
#1924=CARTESIAN_POINT('Ctrl Pts',(-16.9745170477256,-9.,310.674187150777));
#1925=CARTESIAN_POINT('Ctrl Pts',(-16.9338349467122,-9.,307.69587590639));
#1926=CARTESIAN_POINT('Ctrl Pts',(-16.8634487703245,-9.,304.57015716772));
#1927=CARTESIAN_POINT('Ctrl Pts',(-16.7422790149997,-9.,301.348120547886));
#1928=CARTESIAN_POINT('Ctrl Pts',(-16.5359735439045,-9.,298.095070696299));
#1929=CARTESIAN_POINT('Ctrl Pts',(-16.1926929497518,-9.,294.892205598351));
#1930=CARTESIAN_POINT('Ctrl Pts',(-15.6496061172615,-9.,291.82914277586));
#1931=CARTESIAN_POINT('Ctrl Pts',(-14.8403951587419,-9.,288.995763819941));
#1932=CARTESIAN_POINT('Ctrl Pts',(-13.7033484644208,-9.,286.473438815185));
#1933=CARTESIAN_POINT('Ctrl Pts',(-12.1890242800701,-9.,284.326851421562));
#1934=CARTESIAN_POINT('Ctrl Pts',(-10.2723403348262,-9.,282.590975648728));
#1935=CARTESIAN_POINT('Ctrl Pts',(-7.94806288019228,-9.,281.276448102944));
#1936=CARTESIAN_POINT('Ctrl Pts',(-5.76616670029465,-9.,280.560219196132));
#1937=CARTESIAN_POINT('Ctrl Pts',(-3.9517913938126,-9.,280.208504145521));
#1938=CARTESIAN_POINT('Ctrl Pts',(-2.66368424066569,-9.,280.055862403662));
#1939=CARTESIAN_POINT('Ctrl Pts',(-1.60000000000001,-9.,279.966331939052));
#1940=CARTESIAN_POINT('Ctrl Pts',(-1.20000000000001,-9.,279.932663878104));
#1941=CARTESIAN_POINT('Ctrl Pts',(-0.800000000000013,-9.,279.898995817156));
#1942=CARTESIAN_POINT('Ctrl Pts',(-0.400000000000013,-9.,279.865327756209));
#1943=CARTESIAN_POINT('Ctrl Pts',(-2.04350425470068E-14,-9.,279.831659695261));
#1944=CARTESIAN_POINT('Origin',(2.,9.,302.));
#1945=CARTESIAN_POINT('',(15.,9.,316.));
#1946=CARTESIAN_POINT('Ctrl Pts',(-8.59312621059871E-14,9.,281.838731806122));
#1947=CARTESIAN_POINT('Ctrl Pts',(0.610750952817164,9.,281.890138806881));
#1948=CARTESIAN_POINT('Ctrl Pts',(1.22150190563442,9.,281.941545807639));
#1949=CARTESIAN_POINT('Ctrl Pts',(1.8322528584517,9.,281.992952808398));
#1950=CARTESIAN_POINT('Ctrl Pts',(1.88839473154122,9.,281.99767827841));
#1951=CARTESIAN_POINT('Ctrl Pts',(1.94431052069477,9.,282.002590971222));
#1952=CARTESIAN_POINT('Ctrl Pts',(1.99999999999782,9.,282.007690234858));
#1953=CARTESIAN_POINT('Ctrl Pts',(3.92777602497513,9.,282.18420900116));
#1954=CARTESIAN_POINT('Ctrl Pts',(5.58089918248363,9.,282.584441583133));
#1955=CARTESIAN_POINT('Ctrl Pts',(6.96718239188881,9.,283.179505866003));
#1956=CARTESIAN_POINT('Ctrl Pts',(9.62598372131269,9.,284.320800585332));
#1957=CARTESIAN_POINT('Ctrl Pts',(11.3428854490917,9.,286.13723179047));
#1958=CARTESIAN_POINT('Ctrl Pts',(12.5329121501934,9.,288.887907445925));
#1959=CARTESIAN_POINT('Ctrl Pts',(14.3613339472215,9.,293.114195242939));
#1960=CARTESIAN_POINT('Ctrl Pts',(14.7151010160305,9.,299.547166753218));
#1961=CARTESIAN_POINT('Ctrl Pts',(14.8743203079702,9.,305.389849883143));
#1962=CARTESIAN_POINT('Ctrl Pts',(14.9804665025967,9.,309.284971969759));
#1963=CARTESIAN_POINT('Ctrl Pts',(15.,9.,312.917218954967));
#1964=CARTESIAN_POINT('Ctrl Pts',(15.,9.,316.));
#1965=CARTESIAN_POINT('',(15.,9.,324.));
#1966=CARTESIAN_POINT('',(15.,9.,324.));
#1967=CARTESIAN_POINT('',(17.,9.,324.));
#1968=CARTESIAN_POINT('',(-13.,9.,324.));
#1969=CARTESIAN_POINT('',(17.,9.,316.));
#1970=CARTESIAN_POINT('',(17.,9.,324.));
#1971=CARTESIAN_POINT('Ctrl Pts',(7.73686670285656E-15,9.,279.831659695261));
#1972=CARTESIAN_POINT('Ctrl Pts',(0.400000000000004,9.,279.865327756209));
#1973=CARTESIAN_POINT('Ctrl Pts',(0.800000000000005,9.,279.898995817156));
#1974=CARTESIAN_POINT('Ctrl Pts',(1.2,9.,279.932663878104));
#1975=CARTESIAN_POINT('Ctrl Pts',(1.6,9.,279.966331939052));
#1976=CARTESIAN_POINT('Ctrl Pts',(2.66368424066569,9.,280.055862403662));
#1977=CARTESIAN_POINT('Ctrl Pts',(3.9517913938126,9.,280.208504145521));
#1978=CARTESIAN_POINT('Ctrl Pts',(5.76616670029465,9.,280.560219196132));
#1979=CARTESIAN_POINT('Ctrl Pts',(7.94806288019228,9.,281.276448102944));
#1980=CARTESIAN_POINT('Ctrl Pts',(10.2723403348262,9.,282.590975648728));
#1981=CARTESIAN_POINT('Ctrl Pts',(12.1890242800701,9.,284.326851421562));
#1982=CARTESIAN_POINT('Ctrl Pts',(13.7033484644208,9.,286.473438815185));
#1983=CARTESIAN_POINT('Ctrl Pts',(14.8403951587419,9.,288.995763819941));
#1984=CARTESIAN_POINT('Ctrl Pts',(15.6496061172615,9.,291.82914277586));
#1985=CARTESIAN_POINT('Ctrl Pts',(16.1926929497518,9.,294.892205598351));
#1986=CARTESIAN_POINT('Ctrl Pts',(16.5359735439045,9.,298.095070696299));
#1987=CARTESIAN_POINT('Ctrl Pts',(16.7422790149997,9.,301.348120547886));
#1988=CARTESIAN_POINT('Ctrl Pts',(16.8634487703245,9.,304.57015716772));
#1989=CARTESIAN_POINT('Ctrl Pts',(16.9338349467122,9.,307.69587590639));
#1990=CARTESIAN_POINT('Ctrl Pts',(16.9745170477256,9.,310.674187150777));
#1991=CARTESIAN_POINT('Ctrl Pts',(16.9920318646118,9.,312.909176752281));
#1992=CARTESIAN_POINT('Ctrl Pts',(16.9985513080952,9.,314.491917916066));
#1993=CARTESIAN_POINT('Ctrl Pts',(17.,9.,315.50441646936));
#1994=CARTESIAN_POINT('Ctrl Pts',(17.,9.,316.));
#1995=CARTESIAN_POINT('Origin',(2.,-9.,302.));
#1996=CARTESIAN_POINT('',(17.,-9.,316.));
#1997=CARTESIAN_POINT('Ctrl Pts',(7.73686670285656E-15,-9.,279.831659695261));
#1998=CARTESIAN_POINT('Ctrl Pts',(0.400000000000004,-9.,279.865327756209));
#1999=CARTESIAN_POINT('Ctrl Pts',(0.800000000000005,-9.,279.898995817156));
#2000=CARTESIAN_POINT('Ctrl Pts',(1.2,-9.,279.932663878104));
#2001=CARTESIAN_POINT('Ctrl Pts',(1.6,-9.,279.966331939052));
#2002=CARTESIAN_POINT('Ctrl Pts',(2.66368424066569,-9.,280.055862403662));
#2003=CARTESIAN_POINT('Ctrl Pts',(3.9517913938126,-9.,280.208504145521));
#2004=CARTESIAN_POINT('Ctrl Pts',(5.76616670029465,-9.,280.560219196132));
#2005=CARTESIAN_POINT('Ctrl Pts',(7.94806288019228,-9.,281.276448102944));
#2006=CARTESIAN_POINT('Ctrl Pts',(10.2723403348262,-9.,282.590975648728));
#2007=CARTESIAN_POINT('Ctrl Pts',(12.1890242800701,-9.,284.326851421562));
#2008=CARTESIAN_POINT('Ctrl Pts',(13.7033484644208,-9.,286.473438815185));
#2009=CARTESIAN_POINT('Ctrl Pts',(14.8403951587419,-9.,288.995763819941));
#2010=CARTESIAN_POINT('Ctrl Pts',(15.6496061172615,-9.,291.82914277586));
#2011=CARTESIAN_POINT('Ctrl Pts',(16.1926929497518,-9.,294.892205598351));
#2012=CARTESIAN_POINT('Ctrl Pts',(16.5359735439045,-9.,298.095070696299));
#2013=CARTESIAN_POINT('Ctrl Pts',(16.7422790149997,-9.,301.348120547886));
#2014=CARTESIAN_POINT('Ctrl Pts',(16.8634487703245,-9.,304.57015716772));
#2015=CARTESIAN_POINT('Ctrl Pts',(16.9338349467122,-9.,307.69587590639));
#2016=CARTESIAN_POINT('Ctrl Pts',(16.9745170477256,-9.,310.674187150777));
#2017=CARTESIAN_POINT('Ctrl Pts',(16.9920318646118,-9.,312.909176752281));
#2018=CARTESIAN_POINT('Ctrl Pts',(16.9985513080952,-9.,314.491917916066));
#2019=CARTESIAN_POINT('Ctrl Pts',(17.,-9.,315.50441646936));
#2020=CARTESIAN_POINT('Ctrl Pts',(17.,-9.,316.));
#2021=CARTESIAN_POINT('',(17.,-9.,324.));
#2022=CARTESIAN_POINT('',(17.,-9.,324.));
#2023=CARTESIAN_POINT('',(15.,-9.,324.));
#2024=CARTESIAN_POINT('',(-13.,-9.,324.));
#2025=CARTESIAN_POINT('',(15.,-9.,316.));
#2026=CARTESIAN_POINT('',(15.,-9.,324.));
#2027=CARTESIAN_POINT('Ctrl Pts',(15.,-9.,316.));
#2028=CARTESIAN_POINT('Ctrl Pts',(15.,-9.,312.917218954967));
#2029=CARTESIAN_POINT('Ctrl Pts',(14.9804665025967,-9.,309.284971969759));
#2030=CARTESIAN_POINT('Ctrl Pts',(14.8743203079702,-9.,305.389849883143));
#2031=CARTESIAN_POINT('Ctrl Pts',(14.7151010160305,-9.,299.547166753218));
#2032=CARTESIAN_POINT('Ctrl Pts',(14.3613339472215,-9.,293.114195242939));
#2033=CARTESIAN_POINT('Ctrl Pts',(12.5329121501934,-9.,288.887907445925));
#2034=CARTESIAN_POINT('Ctrl Pts',(11.3428854490917,-9.,286.13723179047));
#2035=CARTESIAN_POINT('Ctrl Pts',(9.62598372131269,-9.,284.320800585332));
#2036=CARTESIAN_POINT('Ctrl Pts',(6.96718239188881,-9.,283.179505866003));
#2037=CARTESIAN_POINT('Ctrl Pts',(5.58089918248363,-9.,282.584441583133));
#2038=CARTESIAN_POINT('Ctrl Pts',(3.92777602497513,-9.,282.18420900116));
#2039=CARTESIAN_POINT('Ctrl Pts',(1.99999999999782,-9.,282.007690234858));
#2040=CARTESIAN_POINT('Ctrl Pts',(1.94431052069477,-9.,282.002590971222));
#2041=CARTESIAN_POINT('Ctrl Pts',(1.88839473154122,-9.,281.99767827841));
#2042=CARTESIAN_POINT('Ctrl Pts',(1.8322528584517,-9.,281.992952808398));
#2043=CARTESIAN_POINT('Ctrl Pts',(1.22150190563442,-9.,281.941545807639));
#2044=CARTESIAN_POINT('Ctrl Pts',(0.610750952817164,-9.,281.890138806881));
#2045=CARTESIAN_POINT('Ctrl Pts',(-8.59312621059871E-14,-9.,281.838731806122));
#2046=CARTESIAN_POINT('Ctrl Pts',(17.,-9.,316.));
#2047=CARTESIAN_POINT('Ctrl Pts',(17.,12.6,316.));
#2048=CARTESIAN_POINT('Ctrl Pts',(17.,-9.,315.50441646936));
#2049=CARTESIAN_POINT('Ctrl Pts',(17.,12.6,315.50441646936));
#2050=CARTESIAN_POINT('Ctrl Pts',(16.9985513080952,-9.,314.491917916066));
#2051=CARTESIAN_POINT('Ctrl Pts',(16.9985513080952,12.6,314.491917916066));
#2052=CARTESIAN_POINT('Ctrl Pts',(16.9920318646118,-9.,312.909176752281));
#2053=CARTESIAN_POINT('Ctrl Pts',(16.9920318646118,12.6,312.909176752281));
#2054=CARTESIAN_POINT('Ctrl Pts',(16.9745170477256,-9.,310.674187150777));
#2055=CARTESIAN_POINT('Ctrl Pts',(16.9745170477256,12.6,310.674187150777));
#2056=CARTESIAN_POINT('Ctrl Pts',(16.9338349467122,-9.,307.69587590639));
#2057=CARTESIAN_POINT('Ctrl Pts',(16.9338349467122,12.6,307.69587590639));
#2058=CARTESIAN_POINT('Ctrl Pts',(16.8634487703245,-9.,304.57015716772));
#2059=CARTESIAN_POINT('Ctrl Pts',(16.8634487703245,12.6,304.57015716772));
#2060=CARTESIAN_POINT('Ctrl Pts',(16.7422790149997,-9.,301.348120547886));
#2061=CARTESIAN_POINT('Ctrl Pts',(16.7422790149997,12.6,301.348120547886));
#2062=CARTESIAN_POINT('Ctrl Pts',(16.5359735439045,-9.,298.095070696299));
#2063=CARTESIAN_POINT('Ctrl Pts',(16.5359735439045,12.6,298.095070696299));
#2064=CARTESIAN_POINT('Ctrl Pts',(16.1926929497518,-9.,294.892205598351));
#2065=CARTESIAN_POINT('Ctrl Pts',(16.1926929497518,12.6,294.892205598351));
#2066=CARTESIAN_POINT('Ctrl Pts',(15.6496061172615,-9.,291.82914277586));
#2067=CARTESIAN_POINT('Ctrl Pts',(15.6496061172615,12.6,291.82914277586));
#2068=CARTESIAN_POINT('Ctrl Pts',(14.8403951587419,-9.,288.995763819941));
#2069=CARTESIAN_POINT('Ctrl Pts',(14.8403951587419,12.6,288.995763819941));
#2070=CARTESIAN_POINT('Ctrl Pts',(13.7033484644208,-9.,286.473438815185));
#2071=CARTESIAN_POINT('Ctrl Pts',(13.7033484644208,12.6,286.473438815185));
#2072=CARTESIAN_POINT('Ctrl Pts',(12.1890242800701,-9.,284.326851421562));
#2073=CARTESIAN_POINT('Ctrl Pts',(12.1890242800701,12.6,284.326851421562));
#2074=CARTESIAN_POINT('Ctrl Pts',(10.2723403348262,-9.,282.590975648728));
#2075=CARTESIAN_POINT('Ctrl Pts',(10.2723403348262,12.6,282.590975648728));
#2076=CARTESIAN_POINT('Ctrl Pts',(7.94806288019228,-9.,281.276448102944));
#2077=CARTESIAN_POINT('Ctrl Pts',(7.94806288019228,12.6,281.276448102944));
#2078=CARTESIAN_POINT('Ctrl Pts',(5.76616670029465,-9.,280.560219196132));
#2079=CARTESIAN_POINT('Ctrl Pts',(5.76616670029465,12.6,280.560219196132));
#2080=CARTESIAN_POINT('Ctrl Pts',(3.9517913938126,-9.,280.208504145521));
#2081=CARTESIAN_POINT('Ctrl Pts',(3.9517913938126,12.6,280.208504145521));
#2082=CARTESIAN_POINT('Ctrl Pts',(2.66368424066569,-9.,280.055862403662));
#2083=CARTESIAN_POINT('Ctrl Pts',(2.66368424066569,12.6,280.055862403662));
#2084=CARTESIAN_POINT('Ctrl Pts',(2.,-9.,280.));
#2085=CARTESIAN_POINT('Ctrl Pts',(2.,12.6,280.));
#2086=CARTESIAN_POINT('Ctrl Pts',(1.,-9.,279.91582984763));
#2087=CARTESIAN_POINT('Ctrl Pts',(1.,12.6,279.91582984763));
#2088=CARTESIAN_POINT('Ctrl Pts',(-1.11022302462516E-15,-9.,279.831659695261));
#2089=CARTESIAN_POINT('Ctrl Pts',(-1.11022302462516E-15,12.6,279.831659695261));
#2090=CARTESIAN_POINT('Ctrl Pts',(-1.,-9.,279.747489542891));
#2091=CARTESIAN_POINT('Ctrl Pts',(-1.,12.6,279.747489542891));
#2092=CARTESIAN_POINT('Ctrl Pts',(-2.,-9.,279.663319390522));
#2093=CARTESIAN_POINT('Ctrl Pts',(-2.,12.6,279.663319390522));
#2094=CARTESIAN_POINT('Ctrl Pts',(-3.,-9.,279.579149238152));
#2095=CARTESIAN_POINT('Ctrl Pts',(-3.,12.6,279.579149238152));
#2096=CARTESIAN_POINT('',(17.,0.,316.));
#2097=CARTESIAN_POINT('Origin',(17.,0.,324.));
#2098=CARTESIAN_POINT('',(17.,0.,324.));
#2099=CARTESIAN_POINT('Origin',(15.,0.,324.));
#2100=CARTESIAN_POINT('',(15.,0.,324.));
#2101=CARTESIAN_POINT('Origin',(15.,0.,316.));
#2102=CARTESIAN_POINT('',(15.,0.,316.));
#2103=CARTESIAN_POINT('Ctrl Pts',(-3.46055768059205,-9.01917151683795,281.547456138864));
#2104=CARTESIAN_POINT('Ctrl Pts',(-3.46055768059205,12.6038343033676,281.547456138864));
#2105=CARTESIAN_POINT('Ctrl Pts',(-1.69628750091079,-9.01917151683795,281.695955028708));
#2106=CARTESIAN_POINT('Ctrl Pts',(-1.69628750091079,12.6038343033676,281.695955028708));
#2107=CARTESIAN_POINT('Ctrl Pts',(0.0679826787703758,-9.01917151683795,
281.844453918553));
#2108=CARTESIAN_POINT('Ctrl Pts',(0.0679826787703758,12.6038343033676,281.844453918553));
#2109=CARTESIAN_POINT('Ctrl Pts',(1.8322528584517,-9.01917151683795,281.992952808398));
#2110=CARTESIAN_POINT('Ctrl Pts',(1.8322528584517,12.6038343033676,281.992952808398));
#2111=CARTESIAN_POINT('Ctrl Pts',(1.88839473154122,-9.01917151683795,281.99767827841));
#2112=CARTESIAN_POINT('Ctrl Pts',(1.88839473154122,12.6038343033676,281.99767827841));
#2113=CARTESIAN_POINT('Ctrl Pts',(1.94431052069477,-9.01917151683795,282.002590971222));
#2114=CARTESIAN_POINT('Ctrl Pts',(1.94431052069477,12.6038343033676,282.002590971222));
#2115=CARTESIAN_POINT('Ctrl Pts',(1.99999999999782,-9.01917151683795,282.007690234858));
#2116=CARTESIAN_POINT('Ctrl Pts',(1.99999999999782,12.6038343033676,282.007690234858));
#2117=CARTESIAN_POINT('Ctrl Pts',(3.92777602497513,-9.01917151683795,282.18420900116));
#2118=CARTESIAN_POINT('Ctrl Pts',(3.92777602497513,12.6038343033676,282.18420900116));
#2119=CARTESIAN_POINT('Ctrl Pts',(5.58089918248363,-9.01917151683795,282.584441583133));
#2120=CARTESIAN_POINT('Ctrl Pts',(5.58089918248363,12.6038343033676,282.584441583133));
#2121=CARTESIAN_POINT('Ctrl Pts',(6.96718239188881,-9.01917151683795,283.179505866003));
#2122=CARTESIAN_POINT('Ctrl Pts',(6.96718239188881,12.6038343033676,283.179505866003));
#2123=CARTESIAN_POINT('Ctrl Pts',(9.62598372131269,-9.01917151683795,284.320800585332));
#2124=CARTESIAN_POINT('Ctrl Pts',(9.62598372131269,12.6038343033676,284.320800585332));
#2125=CARTESIAN_POINT('Ctrl Pts',(11.3428854490917,-9.01917151683795,286.13723179047));
#2126=CARTESIAN_POINT('Ctrl Pts',(11.3428854490917,12.6038343033676,286.13723179047));
#2127=CARTESIAN_POINT('Ctrl Pts',(12.5329121501934,-9.01917151683795,288.887907445925));
#2128=CARTESIAN_POINT('Ctrl Pts',(12.5329121501934,12.6038343033676,288.887907445925));
#2129=CARTESIAN_POINT('Ctrl Pts',(14.3613339472215,-9.01917151683795,293.114195242939));
#2130=CARTESIAN_POINT('Ctrl Pts',(14.3613339472215,12.6038343033676,293.114195242939));
#2131=CARTESIAN_POINT('Ctrl Pts',(14.7151010160305,-9.01917151683795,299.547166753218));
#2132=CARTESIAN_POINT('Ctrl Pts',(14.7151010160305,12.6038343033676,299.547166753218));
#2133=CARTESIAN_POINT('Ctrl Pts',(14.8743203079702,-9.01917151683795,305.389849883143));
#2134=CARTESIAN_POINT('Ctrl Pts',(14.8743203079702,12.6038343033676,305.389849883143));
#2135=CARTESIAN_POINT('Ctrl Pts',(14.9804665025967,-9.01917151683795,309.284971969759));
#2136=CARTESIAN_POINT('Ctrl Pts',(14.9804665025967,12.6038343033676,309.284971969759));
#2137=CARTESIAN_POINT('Ctrl Pts',(15.,-9.01917151683795,312.917218954967));
#2138=CARTESIAN_POINT('Ctrl Pts',(15.,12.6038343033676,312.917218954967));
#2139=CARTESIAN_POINT('Ctrl Pts',(15.,-9.01917151683795,316.));
#2140=CARTESIAN_POINT('Ctrl Pts',(15.,12.6038343033676,316.));
#3136=UNCERTAINTY_MEASURE_WITH_UNIT(LENGTH_MEASURE(0.01),#3155,
'DISTANCE_ACCURACY_VALUE',
'Maximum model space distance between geometric entities at asserted c
onnectivities');
#3143=UNCERTAINTY_MEASURE_WITH_UNIT(LENGTH_MEASURE(0.01),#3155,
'DISTANCE_ACCURACY_VALUE',
'Maximum model space distance between geometric entities at asserted c
onnectivities');
#3147=(
GEOMETRIC_REPRESENTATION_CONTEXT(3)
GLOBAL_UNCERTAINTY_ASSIGNED_CONTEXT((#3136))
GLOBAL_UNIT_ASSIGNED_CONTEXT((#3155,#3157,#3158))
REPRESENTATION_CONTEXT('','3D')
);
#3154=(
GEOMETRIC_REPRESENTATION_CONTEXT(3)
GLOBAL_UNCERTAINTY_ASSIGNED_CONTEXT((#3143))
GLOBAL_UNIT_ASSIGNED_CONTEXT((#3155,#3157,#3158))
REPRESENTATION_CONTEXT('','3D')
);
#3155=(
LENGTH_UNIT()
NAMED_UNIT(*)
SI_UNIT(.MILLI.,.METRE.)
);
#3157=(
NAMED_UNIT(*)
PLANE_ANGLE_UNIT()
SI_UNIT($,.RADIAN.)
);
#3158=(
NAMED_UNIT(*)
SI_UNIT($,.STERADIAN.)
SOLID_ANGLE_UNIT()
);
#3162=SHAPE_DEFINITION_REPRESENTATION(#3172,#3191);
#3172=PRODUCT_DEFINITION_SHAPE('',$,#3202);
#3191=SHAPE_REPRESENTATION('',(#1212),#3147);
#3198=PRODUCT_DEFINITION_CONTEXT('part definition',#3230,'design');
#3202=PRODUCT_DEFINITION('Spring_02','Spring_02',#3212,#3198);
#3212=PRODUCT_DEFINITION_FORMATION('',$,#3235);
#3230=APPLICATION_CONTEXT(
'Core Data for Automotive Mechanical Design Process');
#3231=PRODUCT_CONTEXT('part definition',#3230,'mechanical');
#3235=PRODUCT('Spring_02','Spring_02',$,(#3231));
#3243=PRESENTATION_STYLE_ASSIGNMENT((#3245));
#3245=SURFACE_STYLE_USAGE(.BOTH.,#3247);
#3247=SURFACE_SIDE_STYLE('',(#3249));
#3249=SURFACE_STYLE_FILL_AREA(#3251);
#3251=FILL_AREA_STYLE('Opaque(160,160,160)',(#3253));
#3253=FILL_AREA_STYLE_COLOUR('Opaque(160,160,160)',#3255);
#3255=COLOUR_RGB('Opaque(160,160,160)', 0.09019608, 0.27058824, 0.51372549);
ENDSEC;
END-ISO-10303-21;
